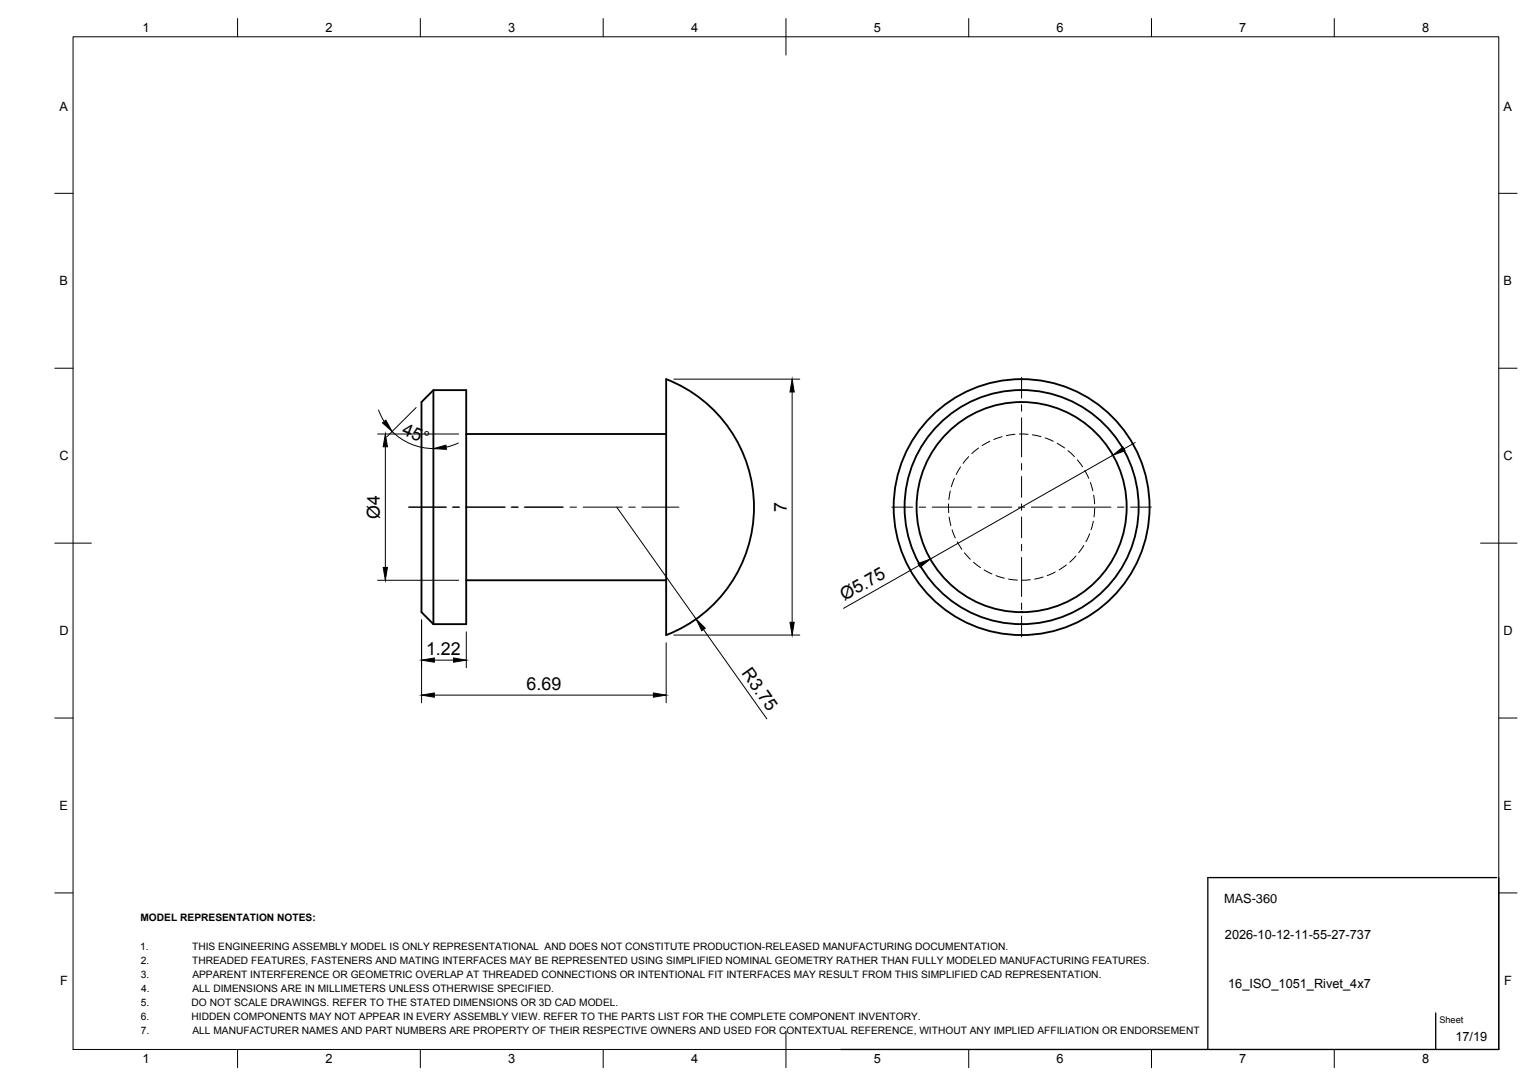
ISO-10303-21;
HEADER;
/* Generated by software containing ST-Developer
 * from STEP Tools, Inc. (www.steptools.com) 
 */

FILE_DESCRIPTION(
/* description */ (''),
/* implementation_level */ '2;1');

FILE_NAME(
/* name */ '16_ISO_1051_Rivet_4x7.step',
/* time_stamp */ '2026-11-04T18:53:29-08:00',
/* author */ (''),
/* organization */ (''),
/* preprocessor_version */ 'ST-DEVELOPER v20.2',
/* originating_system */ 'Autodesk Translation Framework v15.17.0.0',
/* authorisation */ '');

FILE_SCHEMA (('AUTOMOTIVE_DESIGN { 1 0 10303 214 3 1 1 }'));
ENDSEC;

DATA;
#10=MECHANICAL_DESIGN_GEOMETRIC_PRESENTATION_REPRESENTATION('',(#1343),#100031);
#225=SPHERICAL_SURFACE('',#22476,3.75208333333333);
#248=CONICAL_SURFACE('',#22486,3.0368,0.785398163397448);
#1173=CIRCLE('',#22477,3.5);
#1174=CIRCLE('',#22479,2.);
#1175=CIRCLE('',#22481,2.);
#1176=CIRCLE('',#22483,3.2);
#1177=CIRCLE('',#22485,3.2);
#1178=CIRCLE('',#22487,2.8736);
#1307=SHAPE_REPRESENTATION_RELATIONSHIP('SRR','None',#100117,#1325);
#1325=ADVANCED_BREP_SHAPE_REPRESENTATION('',(#1361),#100029);
#1343=STYLED_ITEM('',(#100204),#1361);
#1361=MANIFOLD_SOLID_BREP('Body1',#20133);
#1689=PLANE('',#22478);
#1690=PLANE('',#22482);
#1691=PLANE('',#22488);
#1808=FACE_BOUND('',#7444,.T.);
#1809=FACE_BOUND('',#7447,.T.);
#3262=LINE('',#99937,#4549);
#3263=LINE('',#99944,#4550);
#3264=LINE('',#99947,#4551);
#4549=VECTOR('',#28103,2.);
#4550=VECTOR('',#28112,3.2);
#4551=VECTOR('',#28115,3.0368);
#5023=CYLINDRICAL_SURFACE('',#22480,2.);
#5024=CYLINDRICAL_SURFACE('',#22484,3.2);
#6171=FACE_OUTER_BOUND('',#7442,.T.);
#6172=FACE_OUTER_BOUND('',#7443,.T.);
#6173=FACE_OUTER_BOUND('',#7445,.T.);
#6174=FACE_OUTER_BOUND('',#7446,.T.);
#6175=FACE_OUTER_BOUND('',#7448,.T.);
#6176=FACE_OUTER_BOUND('',#7449,.T.);
#6177=FACE_OUTER_BOUND('',#7450,.T.);
#7442=EDGE_LOOP('',(#18819));
#7443=EDGE_LOOP('',(#18820));
#7444=EDGE_LOOP('',(#18821));
#7445=EDGE_LOOP('',(#18822,#18823,#18824,#18825));
#7446=EDGE_LOOP('',(#18826));
#7447=EDGE_LOOP('',(#18827));
#7448=EDGE_LOOP('',(#18828,#18829,#18830,#18831));
#7449=EDGE_LOOP('',(#18832,#18833,#18834,#18835));
#7450=EDGE_LOOP('',(#18836));
#9914=VERTEX_POINT('',#99929);
#9915=VERTEX_POINT('',#99932);
#9916=VERTEX_POINT('',#99935);
#9917=VERTEX_POINT('',#99939);
#9918=VERTEX_POINT('',#99942);
#9919=VERTEX_POINT('',#99946);
#12884=EDGE_CURVE('',#9914,#9914,#1173,.T.);
#12885=EDGE_CURVE('',#9915,#9915,#1174,.T.);
#12886=EDGE_CURVE('',#9916,#9916,#1175,.T.);
#12887=EDGE_CURVE('',#9916,#9915,#3262,.T.);
#12888=EDGE_CURVE('',#9917,#9917,#1176,.T.);
#12889=EDGE_CURVE('',#9918,#9918,#1177,.T.);
#12890=EDGE_CURVE('',#9918,#9917,#3263,.T.);
#12891=EDGE_CURVE('',#9918,#9919,#3264,.T.);
#12892=EDGE_CURVE('',#9919,#9919,#1178,.T.);
#18819=ORIENTED_EDGE('',*,*,#12884,.F.);
#18820=ORIENTED_EDGE('',*,*,#12884,.T.);
#18821=ORIENTED_EDGE('',*,*,#12885,.F.);
#18822=ORIENTED_EDGE('',*,*,#12886,.F.);
#18823=ORIENTED_EDGE('',*,*,#12887,.T.);
#18824=ORIENTED_EDGE('',*,*,#12885,.T.);
#18825=ORIENTED_EDGE('',*,*,#12887,.F.);
#18826=ORIENTED_EDGE('',*,*,#12888,.F.);
#18827=ORIENTED_EDGE('',*,*,#12886,.T.);
#18828=ORIENTED_EDGE('',*,*,#12889,.F.);
#18829=ORIENTED_EDGE('',*,*,#12890,.T.);
#18830=ORIENTED_EDGE('',*,*,#12888,.T.);
#18831=ORIENTED_EDGE('',*,*,#12890,.F.);
#18832=ORIENTED_EDGE('',*,*,#12889,.T.);
#18833=ORIENTED_EDGE('',*,*,#12891,.T.);
#18834=ORIENTED_EDGE('',*,*,#12892,.F.);
#18835=ORIENTED_EDGE('',*,*,#12891,.F.);
#18836=ORIENTED_EDGE('',*,*,#12892,.T.);
#20105=ADVANCED_FACE('',(#6171),#225,.T.);
#20106=ADVANCED_FACE('',(#6172,#1808),#1689,.T.);
#20107=ADVANCED_FACE('',(#6173),#5023,.T.);
#20108=ADVANCED_FACE('',(#6174,#1809),#1690,.T.);
#20109=ADVANCED_FACE('',(#6175),#5024,.T.);
#20110=ADVANCED_FACE('',(#6176),#248,.T.);
#20111=ADVANCED_FACE('',(#6177),#1691,.T.);
#20133=CLOSED_SHELL('',(#20105,#20106,#20107,#20108,#20109,#20110,#20111));
#22475=AXIS2_PLACEMENT_3D('',#99927,#28089,#28090);
#22476=AXIS2_PLACEMENT_3D('',#99928,#28091,#28092);
#22477=AXIS2_PLACEMENT_3D('',#99930,#28093,#28094);
#22478=AXIS2_PLACEMENT_3D('',#99931,#28095,#28096);
#22479=AXIS2_PLACEMENT_3D('',#99933,#28097,#28098);
#22480=AXIS2_PLACEMENT_3D('',#99934,#28099,#28100);
#22481=AXIS2_PLACEMENT_3D('',#99936,#28101,#28102);
#22482=AXIS2_PLACEMENT_3D('',#99938,#28104,#28105);
#22483=AXIS2_PLACEMENT_3D('',#99940,#28106,#28107);
#22484=AXIS2_PLACEMENT_3D('',#99941,#28108,#28109);
#22485=AXIS2_PLACEMENT_3D('',#99943,#28110,#28111);
#22486=AXIS2_PLACEMENT_3D('',#99945,#28113,#28114);
#22487=AXIS2_PLACEMENT_3D('',#99948,#28116,#28117);
#22488=AXIS2_PLACEMENT_3D('',#99949,#28118,#28119);
#28089=DIRECTION('axis',(0.,0.,1.));
#28090=DIRECTION('refdir',(1.,0.,0.));
#28091=DIRECTION('center_axis',(-1.18358034829556E-16,-1.16627939375949E-19,
1.));
#28092=DIRECTION('ref_axis',(-0.999999546524734,-0.000952339396609238,-5.91790461132479E-17));
#28093=DIRECTION('center_axis',(1.,0.,0.));
#28094=DIRECTION('ref_axis',(0.,0.,-1.));
#28095=DIRECTION('center_axis',(1.,0.,0.));
#28096=DIRECTION('ref_axis',(0.,0.,-1.));
#28097=DIRECTION('center_axis',(1.,0.,0.));
#28098=DIRECTION('ref_axis',(0.,0.,-1.));
#28099=DIRECTION('center_axis',(1.,0.,0.));
#28100=DIRECTION('ref_axis',(0.,1.,0.));
#28101=DIRECTION('center_axis',(1.,0.,0.));
#28102=DIRECTION('ref_axis',(0.,0.,-1.));
#28103=DIRECTION('',(-1.,0.,0.));
#28104=DIRECTION('center_axis',(-1.,0.,0.));
#28105=DIRECTION('ref_axis',(0.,0.,1.));
#28106=DIRECTION('center_axis',(1.,0.,0.));
#28107=DIRECTION('ref_axis',(0.,0.,-1.));
#28108=DIRECTION('center_axis',(1.,0.,0.));
#28109=DIRECTION('ref_axis',(0.,1.,0.));
#28110=DIRECTION('center_axis',(1.,0.,0.));
#28111=DIRECTION('ref_axis',(0.,0.,-1.));
#28112=DIRECTION('',(-1.,0.,0.));
#28113=DIRECTION('center_axis',(-1.,0.,0.));
#28114=DIRECTION('ref_axis',(0.,1.,0.));
#28115=DIRECTION('',(0.707106781186548,0.707106781186547,-8.65956056235493E-17));
#28116=DIRECTION('center_axis',(1.,0.,0.));
#28117=DIRECTION('ref_axis',(0.,0.,-1.));
#28118=DIRECTION('center_axis',(1.,0.,0.));
#28119=DIRECTION('ref_axis',(0.,0.,-1.));
#99927=CARTESIAN_POINT('',(0.,0.,0.));
#99928=CARTESIAN_POINT('Origin',(1.35208333333333,-4.16333634234434E-16,
0.));
#99929=CARTESIAN_POINT('',(0.,3.5,0.));
#99930=CARTESIAN_POINT('Origin',(0.,0.,0.));
#99931=CARTESIAN_POINT('Origin',(0.,2.,0.));
#99932=CARTESIAN_POINT('',(0.,-2.,-2.44929359829471E-16));
#99933=CARTESIAN_POINT('Origin',(0.,0.,0.));
#99934=CARTESIAN_POINT('Origin',(2.7336,0.,0.));
#99935=CARTESIAN_POINT('',(5.4672,-2.,-2.44929359829471E-16));
#99936=CARTESIAN_POINT('Origin',(5.4672,0.,0.));
#99937=CARTESIAN_POINT('',(2.7336,-2.,-2.44929359829471E-16));
#99938=CARTESIAN_POINT('Origin',(5.4672,3.2,0.));
#99939=CARTESIAN_POINT('',(5.4672,-3.2,-3.91886975727153E-16));
#99940=CARTESIAN_POINT('Origin',(5.4672,0.,0.));
#99941=CARTESIAN_POINT('Origin',(5.916,0.,0.));
#99942=CARTESIAN_POINT('',(6.3648,-3.2,-3.91886975727153E-16));
#99943=CARTESIAN_POINT('Origin',(6.3648,0.,0.));
#99944=CARTESIAN_POINT('',(5.916,-3.2,-3.91886975727153E-16));
#99945=CARTESIAN_POINT('Origin',(6.528,0.,0.));
#99946=CARTESIAN_POINT('',(6.6912,-2.8736,-3.51914504202983E-16));
#99947=CARTESIAN_POINT('',(6.528,-3.0368,3.71900739965068E-16));
#99948=CARTESIAN_POINT('Origin',(6.6912,0.,0.));
#99949=CARTESIAN_POINT('Origin',(6.6912,0.,0.));
#100009=UNCERTAINTY_MEASURE_WITH_UNIT(LENGTH_MEASURE(0.01),#100032,
'DISTANCE_ACCURACY_VALUE',
'Maximum model space distance between geometric entities at asserted c
onnectivities');
#100011=UNCERTAINTY_MEASURE_WITH_UNIT(LENGTH_MEASURE(0.01),#100032,
'DISTANCE_ACCURACY_VALUE',
'Maximum model space distance between geometric entities at asserted c
onnectivities');
#100029=(
GEOMETRIC_REPRESENTATION_CONTEXT(3)
GLOBAL_UNCERTAINTY_ASSIGNED_CONTEXT((#100009))
GLOBAL_UNIT_ASSIGNED_CONTEXT((#100032,#100034,#100035))
REPRESENTATION_CONTEXT('','3D')
);
#100031=(
GEOMETRIC_REPRESENTATION_CONTEXT(3)
GLOBAL_UNCERTAINTY_ASSIGNED_CONTEXT((#100011))
GLOBAL_UNIT_ASSIGNED_CONTEXT((#100032,#100034,#100035))
REPRESENTATION_CONTEXT('','3D')
);
#100032=(
LENGTH_UNIT()
NAMED_UNIT(*)
SI_UNIT(.MILLI.,.METRE.)
);
#100034=(
NAMED_UNIT(*)
PLANE_ANGLE_UNIT()
SI_UNIT($,.RADIAN.)
);
#100035=(
NAMED_UNIT(*)
SI_UNIT($,.STERADIAN.)
SOLID_ANGLE_UNIT()
);
#100053=SHAPE_DEFINITION_REPRESENTATION(#100072,#100117);
#100072=PRODUCT_DEFINITION_SHAPE('',$,#100137);
#100117=SHAPE_REPRESENTATION('',(#22475),#100029);
#100119=PRODUCT_DEFINITION_CONTEXT('part definition',#100178,'design');
#100137=PRODUCT_DEFINITION('2026-10-12-11-55-27-737',
'16_ISO_1051_Rivet_4x7',#100156,#100119);
#100156=PRODUCT_DEFINITION_FORMATION('',$,#100197);
#100178=APPLICATION_CONTEXT(
'Core Data for Automotive Mechanical Design Process');
#100179=PRODUCT_CONTEXT('part definition',#100178,'mechanical');
#100197=PRODUCT('2026-10-12-11-55-27-737','16_ISO_1051_Rivet_4x7',$,(#100179));
#100204=PRESENTATION_STYLE_ASSIGNMENT((#100210));
#100210=SURFACE_STYLE_USAGE(.BOTH.,#100216);
#100216=SURFACE_SIDE_STYLE('',(#100222));
#100222=SURFACE_STYLE_FILL_AREA(#100228);
#100228=FILL_AREA_STYLE('Opaque(97,158,199)',(#100234));
#100234=FILL_AREA_STYLE_COLOUR('Opaque(97,158,199)',#100240);
#100240=COLOUR_RGB('Opaque(97,158,199)',0.380392156862745,0.619607843137255,
0.780392156862745);
ENDSEC;
END-ISO-10303-21;
